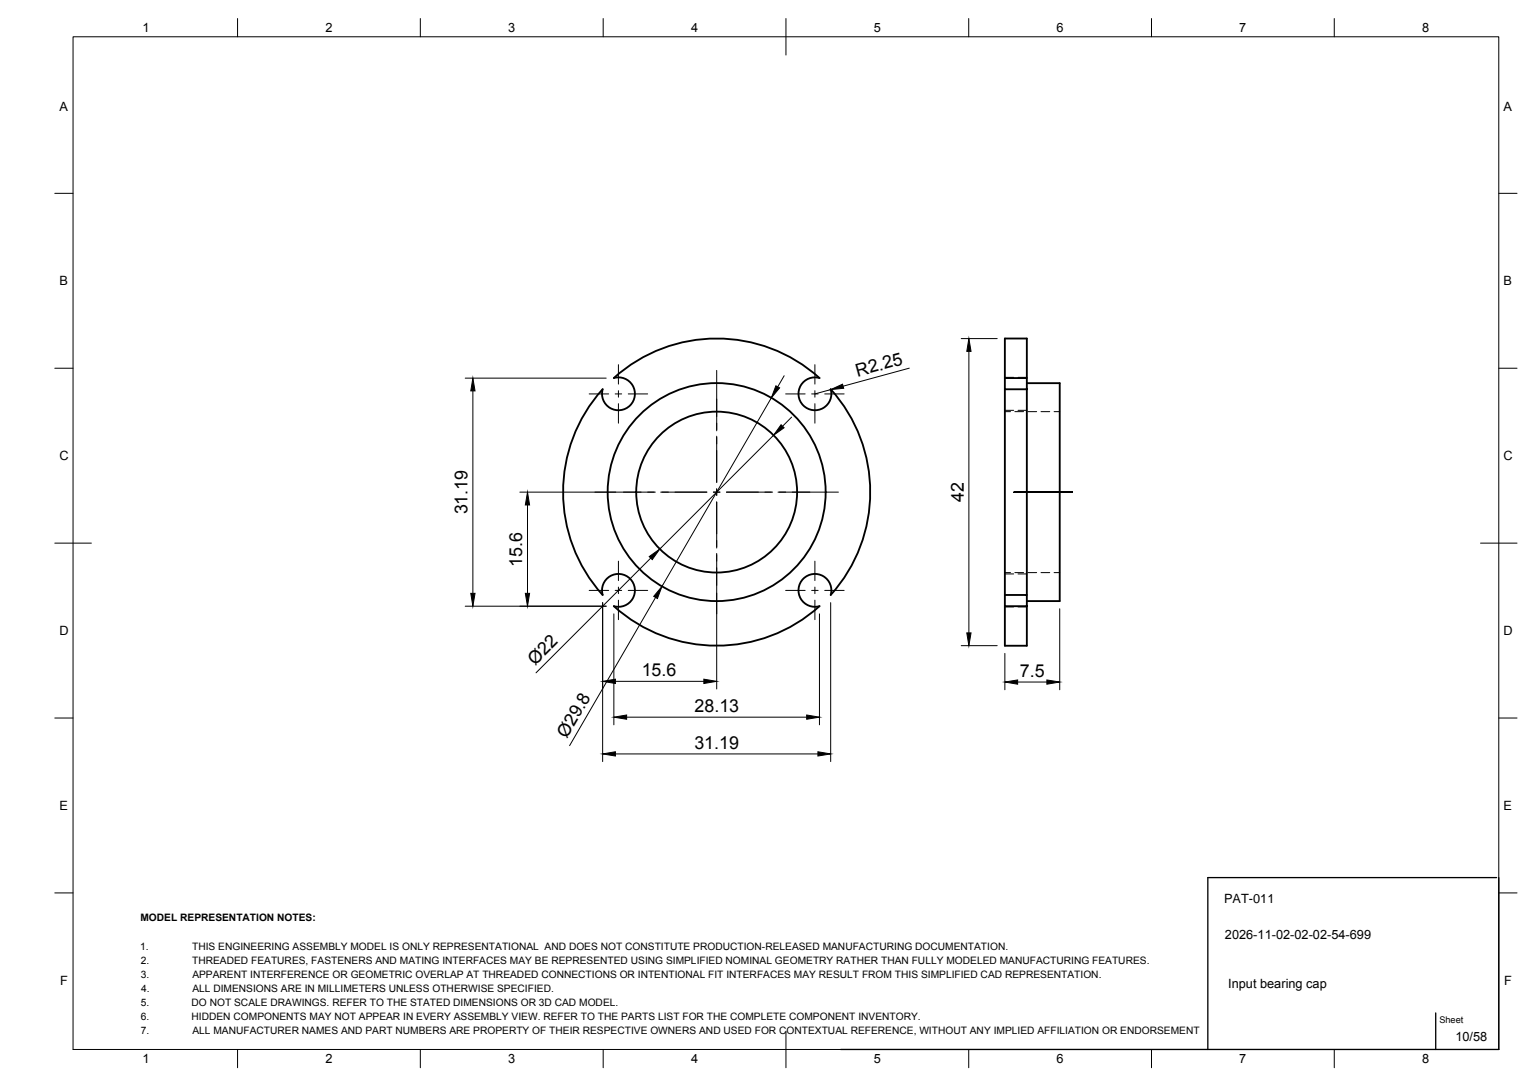
ISO-10303-21;
HEADER;
/* Generated by software containing ST-Developer
 * from STEP Tools, Inc. (www.steptools.com) 
 */

FILE_DESCRIPTION(
/* description */ ('Belt tension measurement rig'),
/* implementation_level */ '2;1');

FILE_NAME(
/* name */ 'Input bearing cap.step',
/* time_stamp */ '2026-10-28T03:24:44-07:00',
/* author */ (''),
/* organization */ (''),
/* preprocessor_version */ 'ST-DEVELOPER v20.2',
/* originating_system */ 'Autodesk Translation Framework v15.17.0.0',
/* authorisation */ '');

FILE_SCHEMA (('AUTOMOTIVE_DESIGN { 1 0 10303 214 3 1 1 }'));
ENDSEC;

DATA;
#10=MECHANICAL_DESIGN_GEOMETRIC_PRESENTATION_REPRESENTATION('',(#697),#23587);
#587=SHAPE_REPRESENTATION_RELATIONSHIP('SRR','None',#23832,#642);
#642=ADVANCED_BREP_SHAPE_REPRESENTATION('',(#767),#23530);
#697=STYLED_ITEM('',(#24211),#767);
#767=MANIFOLD_SOLID_BREP('Body1',#12202);
#863=FACE_BOUND('',#2164,.T.);
#864=FACE_BOUND('',#2171,.T.);
#865=FACE_BOUND('',#2174,.T.);
#1081=PLANE('',#13015);
#1082=PLANE('',#13032);
#1083=PLANE('',#13035);
#1421=FACE_OUTER_BOUND('',#2159,.T.);
#1422=FACE_OUTER_BOUND('',#2160,.T.);
#1423=FACE_OUTER_BOUND('',#2161,.T.);
#1424=FACE_OUTER_BOUND('',#2162,.T.);
#1425=FACE_OUTER_BOUND('',#2163,.T.);
#1426=FACE_OUTER_BOUND('',#2165,.T.);
#1427=FACE_OUTER_BOUND('',#2166,.T.);
#1428=FACE_OUTER_BOUND('',#2167,.T.);
#1429=FACE_OUTER_BOUND('',#2168,.T.);
#1430=FACE_OUTER_BOUND('',#2169,.T.);
#1431=FACE_OUTER_BOUND('',#2170,.T.);
#1432=FACE_OUTER_BOUND('',#2172,.T.);
#1433=FACE_OUTER_BOUND('',#2173,.T.);
#2159=EDGE_LOOP('',(#8208,#8209,#8210,#8211));
#2160=EDGE_LOOP('',(#8212,#8213,#8214,#8215));
#2161=EDGE_LOOP('',(#8216,#8217,#8218,#8219));
#2162=EDGE_LOOP('',(#8220,#8221,#8222,#8223));
#2163=EDGE_LOOP('',(#8224,#8225,#8226,#8227,#8228,#8229,#8230,#8231));
#2164=EDGE_LOOP('',(#8232));
#2165=EDGE_LOOP('',(#8233,#8234,#8235,#8236));
#2166=EDGE_LOOP('',(#8237,#8238,#8239,#8240));
#2167=EDGE_LOOP('',(#8241,#8242,#8243,#8244));
#2168=EDGE_LOOP('',(#8245,#8246,#8247,#8248));
#2169=EDGE_LOOP('',(#8249,#8250,#8251,#8252));
#2170=EDGE_LOOP('',(#8253));
#2171=EDGE_LOOP('',(#8254));
#2172=EDGE_LOOP('',(#8255,#8256,#8257,#8258));
#2173=EDGE_LOOP('',(#8259,#8260,#8261,#8262,#8263,#8264,#8265,#8266));
#2174=EDGE_LOOP('',(#8267));
#3053=LINE('',#18855,#3804);
#3054=LINE('',#18859,#3805);
#3055=LINE('',#18864,#3806);
#3056=LINE('',#18868,#3807);
#3057=LINE('',#18873,#3808);
#3058=LINE('',#18877,#3809);
#3059=LINE('',#18882,#3810);
#3060=LINE('',#18886,#3811);
#3061=LINE('',#18907,#3812);
#3062=LINE('',#18913,#3813);
#3804=VECTOR('',#14858,1.);
#3805=VECTOR('',#14861,1.);
#3806=VECTOR('',#14866,1.);
#3807=VECTOR('',#14869,1.);
#3808=VECTOR('',#14874,1.);
#3809=VECTOR('',#14877,1.);
#3810=VECTOR('',#14882,1.);
#3811=VECTOR('',#14885,1.);
#3812=VECTOR('',#14920,1.49);
#3813=VECTOR('',#14929,1.1);
#4520=CIRCLE('',#13004,0.225);
#4521=CIRCLE('',#13005,0.225);
#4522=CIRCLE('',#13007,0.225);
#4523=CIRCLE('',#13008,0.225);
#4524=CIRCLE('',#13010,0.225);
#4525=CIRCLE('',#13011,0.225);
#4526=CIRCLE('',#13013,0.225);
#4527=CIRCLE('',#13014,0.225);
#4528=CIRCLE('',#13016,2.1);
#4529=CIRCLE('',#13017,2.1);
#4530=CIRCLE('',#13018,2.1);
#4531=CIRCLE('',#13019,2.1);
#4532=CIRCLE('',#13020,1.1);
#4533=CIRCLE('',#13022,2.1);
#4534=CIRCLE('',#13024,2.1);
#4535=CIRCLE('',#13026,2.1);
#4536=CIRCLE('',#13028,2.1);
#4537=CIRCLE('',#13030,1.49);
#4538=CIRCLE('',#13031,1.49);
#4539=CIRCLE('',#13033,1.1);
#5328=VERTEX_POINT('',#18853);
#5329=VERTEX_POINT('',#18854);
#5330=VERTEX_POINT('',#18856);
#5331=VERTEX_POINT('',#18858);
#5332=VERTEX_POINT('',#18862);
#5333=VERTEX_POINT('',#18863);
#5334=VERTEX_POINT('',#18865);
#5335=VERTEX_POINT('',#18867);
#5336=VERTEX_POINT('',#18871);
#5337=VERTEX_POINT('',#18872);
#5338=VERTEX_POINT('',#18874);
#5339=VERTEX_POINT('',#18876);
#5340=VERTEX_POINT('',#18880);
#5341=VERTEX_POINT('',#18881);
#5342=VERTEX_POINT('',#18883);
#5343=VERTEX_POINT('',#18885);
#5344=VERTEX_POINT('',#18893);
#5345=VERTEX_POINT('',#18904);
#5346=VERTEX_POINT('',#18906);
#5347=VERTEX_POINT('',#18910);
#6463=EDGE_CURVE('',#5328,#5329,#3053,.T.);
#6464=EDGE_CURVE('',#5330,#5328,#4520,.T.);
#6465=EDGE_CURVE('',#5331,#5330,#3054,.T.);
#6466=EDGE_CURVE('',#5329,#5331,#4521,.T.);
#6467=EDGE_CURVE('',#5332,#5333,#3055,.T.);
#6468=EDGE_CURVE('',#5334,#5332,#4522,.T.);
#6469=EDGE_CURVE('',#5335,#5334,#3056,.T.);
#6470=EDGE_CURVE('',#5333,#5335,#4523,.T.);
#6471=EDGE_CURVE('',#5336,#5337,#3057,.T.);
#6472=EDGE_CURVE('',#5338,#5336,#4524,.T.);
#6473=EDGE_CURVE('',#5339,#5338,#3058,.T.);
#6474=EDGE_CURVE('',#5337,#5339,#4525,.T.);
#6475=EDGE_CURVE('',#5340,#5341,#3059,.T.);
#6476=EDGE_CURVE('',#5342,#5340,#4526,.T.);
#6477=EDGE_CURVE('',#5343,#5342,#3060,.T.);
#6478=EDGE_CURVE('',#5341,#5343,#4527,.T.);
#6479=EDGE_CURVE('',#5342,#5328,#4528,.T.);
#6480=EDGE_CURVE('',#5338,#5340,#4529,.T.);
#6481=EDGE_CURVE('',#5334,#5336,#4530,.T.);
#6482=EDGE_CURVE('',#5330,#5332,#4531,.T.);
#6483=EDGE_CURVE('',#5344,#5344,#4532,.T.);
#6484=EDGE_CURVE('',#5339,#5341,#4533,.T.);
#6485=EDGE_CURVE('',#5335,#5337,#4534,.T.);
#6486=EDGE_CURVE('',#5343,#5329,#4535,.T.);
#6487=EDGE_CURVE('',#5331,#5333,#4536,.T.);
#6488=EDGE_CURVE('',#5345,#5345,#4537,.T.);
#6489=EDGE_CURVE('',#5345,#5346,#3061,.T.);
#6490=EDGE_CURVE('',#5346,#5346,#4538,.T.);
#6491=EDGE_CURVE('',#5347,#5347,#4539,.T.);
#6492=EDGE_CURVE('',#5347,#5344,#3062,.T.);
#8208=ORIENTED_EDGE('',*,*,#6463,.F.);
#8209=ORIENTED_EDGE('',*,*,#6464,.F.);
#8210=ORIENTED_EDGE('',*,*,#6465,.F.);
#8211=ORIENTED_EDGE('',*,*,#6466,.F.);
#8212=ORIENTED_EDGE('',*,*,#6467,.F.);
#8213=ORIENTED_EDGE('',*,*,#6468,.F.);
#8214=ORIENTED_EDGE('',*,*,#6469,.F.);
#8215=ORIENTED_EDGE('',*,*,#6470,.F.);
#8216=ORIENTED_EDGE('',*,*,#6471,.F.);
#8217=ORIENTED_EDGE('',*,*,#6472,.F.);
#8218=ORIENTED_EDGE('',*,*,#6473,.F.);
#8219=ORIENTED_EDGE('',*,*,#6474,.F.);
#8220=ORIENTED_EDGE('',*,*,#6475,.F.);
#8221=ORIENTED_EDGE('',*,*,#6476,.F.);
#8222=ORIENTED_EDGE('',*,*,#6477,.F.);
#8223=ORIENTED_EDGE('',*,*,#6478,.F.);
#8224=ORIENTED_EDGE('',*,*,#6464,.T.);
#8225=ORIENTED_EDGE('',*,*,#6479,.F.);
#8226=ORIENTED_EDGE('',*,*,#6476,.T.);
#8227=ORIENTED_EDGE('',*,*,#6480,.F.);
#8228=ORIENTED_EDGE('',*,*,#6472,.T.);
#8229=ORIENTED_EDGE('',*,*,#6481,.F.);
#8230=ORIENTED_EDGE('',*,*,#6468,.T.);
#8231=ORIENTED_EDGE('',*,*,#6482,.F.);
#8232=ORIENTED_EDGE('',*,*,#6483,.F.);
#8233=ORIENTED_EDGE('',*,*,#6473,.T.);
#8234=ORIENTED_EDGE('',*,*,#6480,.T.);
#8235=ORIENTED_EDGE('',*,*,#6475,.T.);
#8236=ORIENTED_EDGE('',*,*,#6484,.F.);
#8237=ORIENTED_EDGE('',*,*,#6469,.T.);
#8238=ORIENTED_EDGE('',*,*,#6481,.T.);
#8239=ORIENTED_EDGE('',*,*,#6471,.T.);
#8240=ORIENTED_EDGE('',*,*,#6485,.F.);
#8241=ORIENTED_EDGE('',*,*,#6463,.T.);
#8242=ORIENTED_EDGE('',*,*,#6486,.F.);
#8243=ORIENTED_EDGE('',*,*,#6477,.T.);
#8244=ORIENTED_EDGE('',*,*,#6479,.T.);
#8245=ORIENTED_EDGE('',*,*,#6465,.T.);
#8246=ORIENTED_EDGE('',*,*,#6482,.T.);
#8247=ORIENTED_EDGE('',*,*,#6467,.T.);
#8248=ORIENTED_EDGE('',*,*,#6487,.F.);
#8249=ORIENTED_EDGE('',*,*,#6488,.F.);
#8250=ORIENTED_EDGE('',*,*,#6489,.T.);
#8251=ORIENTED_EDGE('',*,*,#6490,.F.);
#8252=ORIENTED_EDGE('',*,*,#6489,.F.);
#8253=ORIENTED_EDGE('',*,*,#6488,.T.);
#8254=ORIENTED_EDGE('',*,*,#6491,.T.);
#8255=ORIENTED_EDGE('',*,*,#6491,.F.);
#8256=ORIENTED_EDGE('',*,*,#6492,.T.);
#8257=ORIENTED_EDGE('',*,*,#6483,.T.);
#8258=ORIENTED_EDGE('',*,*,#6492,.F.);
#8259=ORIENTED_EDGE('',*,*,#6466,.T.);
#8260=ORIENTED_EDGE('',*,*,#6487,.T.);
#8261=ORIENTED_EDGE('',*,*,#6470,.T.);
#8262=ORIENTED_EDGE('',*,*,#6485,.T.);
#8263=ORIENTED_EDGE('',*,*,#6474,.T.);
#8264=ORIENTED_EDGE('',*,*,#6484,.T.);
#8265=ORIENTED_EDGE('',*,*,#6478,.T.);
#8266=ORIENTED_EDGE('',*,*,#6486,.T.);
#8267=ORIENTED_EDGE('',*,*,#6490,.T.);
#11183=CYLINDRICAL_SURFACE('',#13003,0.225);
#11184=CYLINDRICAL_SURFACE('',#13006,0.225);
#11185=CYLINDRICAL_SURFACE('',#13009,0.225);
#11186=CYLINDRICAL_SURFACE('',#13012,0.225);
#11187=CYLINDRICAL_SURFACE('',#13021,2.1);
#11188=CYLINDRICAL_SURFACE('',#13023,2.1);
#11189=CYLINDRICAL_SURFACE('',#13025,2.1);
#11190=CYLINDRICAL_SURFACE('',#13027,2.1);
#11191=CYLINDRICAL_SURFACE('',#13029,1.49);
#11192=CYLINDRICAL_SURFACE('',#13034,1.1);
#11562=ADVANCED_FACE('',(#1421),#11183,.F.);
#11563=ADVANCED_FACE('',(#1422),#11184,.F.);
#11564=ADVANCED_FACE('',(#1423),#11185,.F.);
#11565=ADVANCED_FACE('',(#1424),#11186,.F.);
#11566=ADVANCED_FACE('',(#1425,#863),#1081,.F.);
#11567=ADVANCED_FACE('',(#1426),#11187,.T.);
#11568=ADVANCED_FACE('',(#1427),#11188,.T.);
#11569=ADVANCED_FACE('',(#1428),#11189,.T.);
#11570=ADVANCED_FACE('',(#1429),#11190,.T.);
#11571=ADVANCED_FACE('',(#1430),#11191,.T.);
#11572=ADVANCED_FACE('',(#1431,#864),#1082,.T.);
#11573=ADVANCED_FACE('',(#1432),#11192,.F.);
#11574=ADVANCED_FACE('',(#1433,#865),#1083,.T.);
#12202=CLOSED_SHELL('',(#11562,#11563,#11564,#11565,#11566,#11567,#11568,
#11569,#11570,#11571,#11572,#11573,#11574));
#13002=AXIS2_PLACEMENT_3D('',#18851,#14854,#14855);
#13003=AXIS2_PLACEMENT_3D('',#18852,#14856,#14857);
#13004=AXIS2_PLACEMENT_3D('',#18857,#14859,#14860);
#13005=AXIS2_PLACEMENT_3D('',#18860,#14862,#14863);
#13006=AXIS2_PLACEMENT_3D('',#18861,#14864,#14865);
#13007=AXIS2_PLACEMENT_3D('',#18866,#14867,#14868);
#13008=AXIS2_PLACEMENT_3D('',#18869,#14870,#14871);
#13009=AXIS2_PLACEMENT_3D('',#18870,#14872,#14873);
#13010=AXIS2_PLACEMENT_3D('',#18875,#14875,#14876);
#13011=AXIS2_PLACEMENT_3D('',#18878,#14878,#14879);
#13012=AXIS2_PLACEMENT_3D('',#18879,#14880,#14881);
#13013=AXIS2_PLACEMENT_3D('',#18884,#14883,#14884);
#13014=AXIS2_PLACEMENT_3D('',#18887,#14886,#14887);
#13015=AXIS2_PLACEMENT_3D('',#18888,#14888,#14889);
#13016=AXIS2_PLACEMENT_3D('',#18889,#14890,#14891);
#13017=AXIS2_PLACEMENT_3D('',#18890,#14892,#14893);
#13018=AXIS2_PLACEMENT_3D('',#18891,#14894,#14895);
#13019=AXIS2_PLACEMENT_3D('',#18892,#14896,#14897);
#13020=AXIS2_PLACEMENT_3D('',#18894,#14898,#14899);
#13021=AXIS2_PLACEMENT_3D('',#18895,#14900,#14901);
#13022=AXIS2_PLACEMENT_3D('',#18896,#14902,#14903);
#13023=AXIS2_PLACEMENT_3D('',#18897,#14904,#14905);
#13024=AXIS2_PLACEMENT_3D('',#18898,#14906,#14907);
#13025=AXIS2_PLACEMENT_3D('',#18899,#14908,#14909);
#13026=AXIS2_PLACEMENT_3D('',#18900,#14910,#14911);
#13027=AXIS2_PLACEMENT_3D('',#18901,#14912,#14913);
#13028=AXIS2_PLACEMENT_3D('',#18902,#14914,#14915);
#13029=AXIS2_PLACEMENT_3D('',#18903,#14916,#14917);
#13030=AXIS2_PLACEMENT_3D('',#18905,#14918,#14919);
#13031=AXIS2_PLACEMENT_3D('',#18908,#14921,#14922);
#13032=AXIS2_PLACEMENT_3D('',#18909,#14923,#14924);
#13033=AXIS2_PLACEMENT_3D('',#18911,#14925,#14926);
#13034=AXIS2_PLACEMENT_3D('',#18912,#14927,#14928);
#13035=AXIS2_PLACEMENT_3D('',#18914,#14930,#14931);
#14854=DIRECTION('axis',(0.,0.,1.));
#14855=DIRECTION('refdir',(1.,0.,0.));
#14856=DIRECTION('center_axis',(0.,1.,0.));
#14857=DIRECTION('ref_axis',(0.707106781186546,0.,0.707106781186549));
#14858=DIRECTION('',(0.,1.,0.));
#14859=DIRECTION('center_axis',(0.,1.,0.));
#14860=DIRECTION('ref_axis',(1.,0.,0.));
#14861=DIRECTION('',(0.,-1.,0.));
#14862=DIRECTION('center_axis',(0.,-1.,0.));
#14863=DIRECTION('ref_axis',(1.,0.,0.));
#14864=DIRECTION('center_axis',(0.,1.,0.));
#14865=DIRECTION('ref_axis',(0.707106781186547,0.,-0.707106781186548));
#14866=DIRECTION('',(0.,1.,0.));
#14867=DIRECTION('center_axis',(0.,1.,0.));
#14868=DIRECTION('ref_axis',(1.,0.,0.));
#14869=DIRECTION('',(0.,-1.,0.));
#14870=DIRECTION('center_axis',(0.,-1.,0.));
#14871=DIRECTION('ref_axis',(1.,0.,0.));
#14872=DIRECTION('center_axis',(0.,1.,0.));
#14873=DIRECTION('ref_axis',(-0.707106781186552,0.,-0.707106781186543));
#14874=DIRECTION('',(0.,1.,0.));
#14875=DIRECTION('center_axis',(0.,1.,0.));
#14876=DIRECTION('ref_axis',(1.,0.,0.));
#14877=DIRECTION('',(0.,-1.,0.));
#14878=DIRECTION('center_axis',(0.,-1.,0.));
#14879=DIRECTION('ref_axis',(1.,0.,0.));
#14880=DIRECTION('center_axis',(0.,1.,0.));
#14881=DIRECTION('ref_axis',(-0.707106781186546,0.,0.707106781186549));
#14882=DIRECTION('',(0.,1.,0.));
#14883=DIRECTION('center_axis',(0.,1.,0.));
#14884=DIRECTION('ref_axis',(1.,0.,0.));
#14885=DIRECTION('',(0.,-1.,0.));
#14886=DIRECTION('center_axis',(0.,-1.,0.));
#14887=DIRECTION('ref_axis',(1.,0.,0.));
#14888=DIRECTION('center_axis',(0.,1.,0.));
#14889=DIRECTION('ref_axis',(1.,0.,0.));
#14890=DIRECTION('center_axis',(0.,1.,0.));
#14891=DIRECTION('ref_axis',(1.,0.,0.));
#14892=DIRECTION('center_axis',(0.,1.,0.));
#14893=DIRECTION('ref_axis',(1.,0.,0.));
#14894=DIRECTION('center_axis',(0.,1.,0.));
#14895=DIRECTION('ref_axis',(1.,0.,0.));
#14896=DIRECTION('center_axis',(0.,1.,0.));
#14897=DIRECTION('ref_axis',(1.,0.,0.));
#14898=DIRECTION('center_axis',(0.,-1.,0.));
#14899=DIRECTION('ref_axis',(1.,0.,0.));
#14900=DIRECTION('center_axis',(0.,1.,0.));
#14901=DIRECTION('ref_axis',(1.,0.,0.));
#14902=DIRECTION('center_axis',(0.,1.,0.));
#14903=DIRECTION('ref_axis',(1.,0.,0.));
#14904=DIRECTION('center_axis',(0.,1.,0.));
#14905=DIRECTION('ref_axis',(1.,0.,0.));
#14906=DIRECTION('center_axis',(0.,1.,0.));
#14907=DIRECTION('ref_axis',(1.,0.,0.));
#14908=DIRECTION('center_axis',(0.,1.,0.));
#14909=DIRECTION('ref_axis',(1.,0.,0.));
#14910=DIRECTION('center_axis',(0.,1.,0.));
#14911=DIRECTION('ref_axis',(1.,0.,0.));
#14912=DIRECTION('center_axis',(0.,1.,0.));
#14913=DIRECTION('ref_axis',(-1.,0.,-1.22464679914735E-16));
#14914=DIRECTION('center_axis',(0.,1.,0.));
#14915=DIRECTION('ref_axis',(1.,0.,0.));
#14916=DIRECTION('center_axis',(0.,1.,0.));
#14917=DIRECTION('ref_axis',(1.,0.,0.));
#14918=DIRECTION('center_axis',(0.,1.,0.));
#14919=DIRECTION('ref_axis',(1.,0.,0.));
#14920=DIRECTION('',(0.,-1.,0.));
#14921=DIRECTION('center_axis',(0.,-1.,0.));
#14922=DIRECTION('ref_axis',(1.,0.,0.));
#14923=DIRECTION('center_axis',(0.,1.,0.));
#14924=DIRECTION('ref_axis',(1.,0.,0.));
#14925=DIRECTION('center_axis',(0.,-1.,0.));
#14926=DIRECTION('ref_axis',(1.,0.,0.));
#14927=DIRECTION('center_axis',(0.,1.,0.));
#14928=DIRECTION('ref_axis',(1.,0.,0.));
#14929=DIRECTION('',(0.,-1.,0.));
#14930=DIRECTION('center_axis',(0.,1.,0.));
#14931=DIRECTION('ref_axis',(1.,0.,0.));
#18851=CARTESIAN_POINT('',(0.,0.,0.));
#18852=CARTESIAN_POINT('Origin',(-1.34350288425444,-2.2,5.65649711574556));
#18853=CARTESIAN_POINT('',(-1.40634555589641,-2.1,5.4404512904656));
#18854=CARTESIAN_POINT('',(-1.40634555589641,-1.8,5.4404512904656));
#18855=CARTESIAN_POINT('',(-1.40634555589641,-2.2,5.4404512904656));
#18856=CARTESIAN_POINT('',(-1.5595487095344,-2.1,5.59365444410359));
#18857=CARTESIAN_POINT('Origin',(-1.34350288425444,-2.1,5.65649711574556));
#18858=CARTESIAN_POINT('',(-1.5595487095344,-1.8,5.59365444410359));
#18859=CARTESIAN_POINT('',(-1.5595487095344,-2.2,5.59365444410359));
#18860=CARTESIAN_POINT('Origin',(-1.34350288425444,-1.8,5.65649711574556));
#18861=CARTESIAN_POINT('Origin',(-1.34350288425444,-2.2,8.34350288425444));
#18862=CARTESIAN_POINT('',(-1.5595487095344,-2.1,8.40634555589641));
#18863=CARTESIAN_POINT('',(-1.5595487095344,-1.8,8.40634555589641));
#18864=CARTESIAN_POINT('',(-1.5595487095344,-2.2,8.40634555589641));
#18865=CARTESIAN_POINT('',(-1.40634555589641,-2.1,8.5595487095344));
#18866=CARTESIAN_POINT('Origin',(-1.34350288425444,-2.1,8.34350288425444));
#18867=CARTESIAN_POINT('',(-1.40634555589641,-1.8,8.5595487095344));
#18868=CARTESIAN_POINT('',(-1.40634555589641,-2.2,8.5595487095344));
#18869=CARTESIAN_POINT('Origin',(-1.34350288425444,-1.8,8.34350288425444));
#18870=CARTESIAN_POINT('Origin',(1.34350288425444,-2.2,8.34350288425444));
#18871=CARTESIAN_POINT('',(1.40634555589641,-2.1,8.5595487095344));
#18872=CARTESIAN_POINT('',(1.40634555589641,-1.8,8.5595487095344));
#18873=CARTESIAN_POINT('',(1.40634555589641,-2.2,8.5595487095344));
#18874=CARTESIAN_POINT('',(1.5595487095344,-2.1,8.40634555589641));
#18875=CARTESIAN_POINT('Origin',(1.34350288425444,-2.1,8.34350288425444));
#18876=CARTESIAN_POINT('',(1.5595487095344,-1.8,8.40634555589641));
#18877=CARTESIAN_POINT('',(1.5595487095344,-2.2,8.40634555589641));
#18878=CARTESIAN_POINT('Origin',(1.34350288425444,-1.8,8.34350288425444));
#18879=CARTESIAN_POINT('Origin',(1.34350288425444,-2.2,5.65649711574556));
#18880=CARTESIAN_POINT('',(1.5595487095344,-2.1,5.59365444410359));
#18881=CARTESIAN_POINT('',(1.5595487095344,-1.8,5.59365444410359));
#18882=CARTESIAN_POINT('',(1.5595487095344,-2.2,5.59365444410359));
#18883=CARTESIAN_POINT('',(1.40634555589641,-2.1,5.4404512904656));
#18884=CARTESIAN_POINT('Origin',(1.34350288425444,-2.1,5.65649711574556));
#18885=CARTESIAN_POINT('',(1.40634555589641,-1.8,5.4404512904656));
#18886=CARTESIAN_POINT('',(1.40634555589641,-2.2,5.4404512904656));
#18887=CARTESIAN_POINT('Origin',(1.34350288425444,-1.8,5.65649711574556));
#18888=CARTESIAN_POINT('Origin',(0.,-2.1,7.));
#18889=CARTESIAN_POINT('Origin',(0.,-2.1,7.));
#18890=CARTESIAN_POINT('Origin',(0.,-2.1,7.));
#18891=CARTESIAN_POINT('Origin',(0.,-2.1,7.));
#18892=CARTESIAN_POINT('Origin',(0.,-2.1,7.));
#18893=CARTESIAN_POINT('',(-1.1,-2.1,7.));
#18894=CARTESIAN_POINT('Origin',(0.,-2.1,7.));
#18895=CARTESIAN_POINT('Origin',(0.,-2.1,7.));
#18896=CARTESIAN_POINT('Origin',(0.,-1.8,7.));
#18897=CARTESIAN_POINT('Origin',(0.,-2.1,7.));
#18898=CARTESIAN_POINT('Origin',(0.,-1.8,7.));
#18899=CARTESIAN_POINT('Origin',(0.,-2.1,7.));
#18900=CARTESIAN_POINT('Origin',(0.,-1.8,7.));
#18901=CARTESIAN_POINT('Origin',(0.,-2.1,7.));
#18902=CARTESIAN_POINT('Origin',(0.,-1.8,7.));
#18903=CARTESIAN_POINT('Origin',(0.,-1.8,7.));
#18904=CARTESIAN_POINT('',(-1.49,-1.35,7.));
#18905=CARTESIAN_POINT('Origin',(0.,-1.35,7.));
#18906=CARTESIAN_POINT('',(-1.49,-1.8,7.));
#18907=CARTESIAN_POINT('',(-1.49,-1.8,7.));
#18908=CARTESIAN_POINT('Origin',(0.,-1.8,7.));
#18909=CARTESIAN_POINT('Origin',(0.,-1.35,7.));
#18910=CARTESIAN_POINT('',(-1.1,-1.35,7.));
#18911=CARTESIAN_POINT('Origin',(0.,-1.35,7.));
#18912=CARTESIAN_POINT('Origin',(0.,-2.1,7.));
#18913=CARTESIAN_POINT('',(-1.1,-2.1,7.));
#18914=CARTESIAN_POINT('Origin',(0.,-1.8,7.));
#23465=UNCERTAINTY_MEASURE_WITH_UNIT(LENGTH_MEASURE(0.001),#23588,
'DISTANCE_ACCURACY_VALUE',
'Maximum model space distance between geometric entities at asserted c
onnectivities');
#23522=UNCERTAINTY_MEASURE_WITH_UNIT(LENGTH_MEASURE(0.001),#23588,
'DISTANCE_ACCURACY_VALUE',
'Maximum model space distance between geometric entities at asserted c
onnectivities');
#23530=(
GEOMETRIC_REPRESENTATION_CONTEXT(3)
GLOBAL_UNCERTAINTY_ASSIGNED_CONTEXT((#23465))
GLOBAL_UNIT_ASSIGNED_CONTEXT((#23588,#23590,#23591))
REPRESENTATION_CONTEXT('','3D')
);
#23587=(
GEOMETRIC_REPRESENTATION_CONTEXT(3)
GLOBAL_UNCERTAINTY_ASSIGNED_CONTEXT((#23522))
GLOBAL_UNIT_ASSIGNED_CONTEXT((#23588,#23590,#23591))
REPRESENTATION_CONTEXT('','3D')
);
#23588=(
LENGTH_UNIT()
NAMED_UNIT(*)
SI_UNIT(.CENTI.,.METRE.)
);
#23590=(
NAMED_UNIT(*)
PLANE_ANGLE_UNIT()
SI_UNIT($,.RADIAN.)
);
#23591=(
NAMED_UNIT(*)
SI_UNIT($,.STERADIAN.)
SOLID_ANGLE_UNIT()
);
#23599=SHAPE_DEFINITION_REPRESENTATION(#23663,#23832);
#23663=PRODUCT_DEFINITION_SHAPE('',$,#23897);
#23832=SHAPE_REPRESENTATION('',(#13002),#23530);
#23889=PRODUCT_DEFINITION_CONTEXT('part definition',#24083,'design');
#23897=PRODUCT_DEFINITION('Input bearing cap','Input bearing cap',#23961,
#23889);
#23961=PRODUCT_DEFINITION_FORMATION('',$,#24092);
#24083=APPLICATION_CONTEXT(
'Core Data for Automotive Mechanical Design Process');
#24084=PRODUCT_CONTEXT('part definition',#24083,'mechanical');
#24092=PRODUCT('Input bearing cap','Input bearing cap',
'Input bearing cap',(#24084));
#24205=COLOUR_RGB('Grey',0.48,0.52,0.57);
#24206=FILL_AREA_STYLE_COLOUR('',#24205);
#24207=FILL_AREA_STYLE('',(#24206));
#24208=SURFACE_STYLE_FILL_AREA(#24207);
#24209=SURFACE_SIDE_STYLE('',(#24208));
#24210=SURFACE_STYLE_USAGE(.BOTH.,#24209);
#24211=PRESENTATION_STYLE_ASSIGNMENT((#24210));
ENDSEC;
END-ISO-10303-21;
